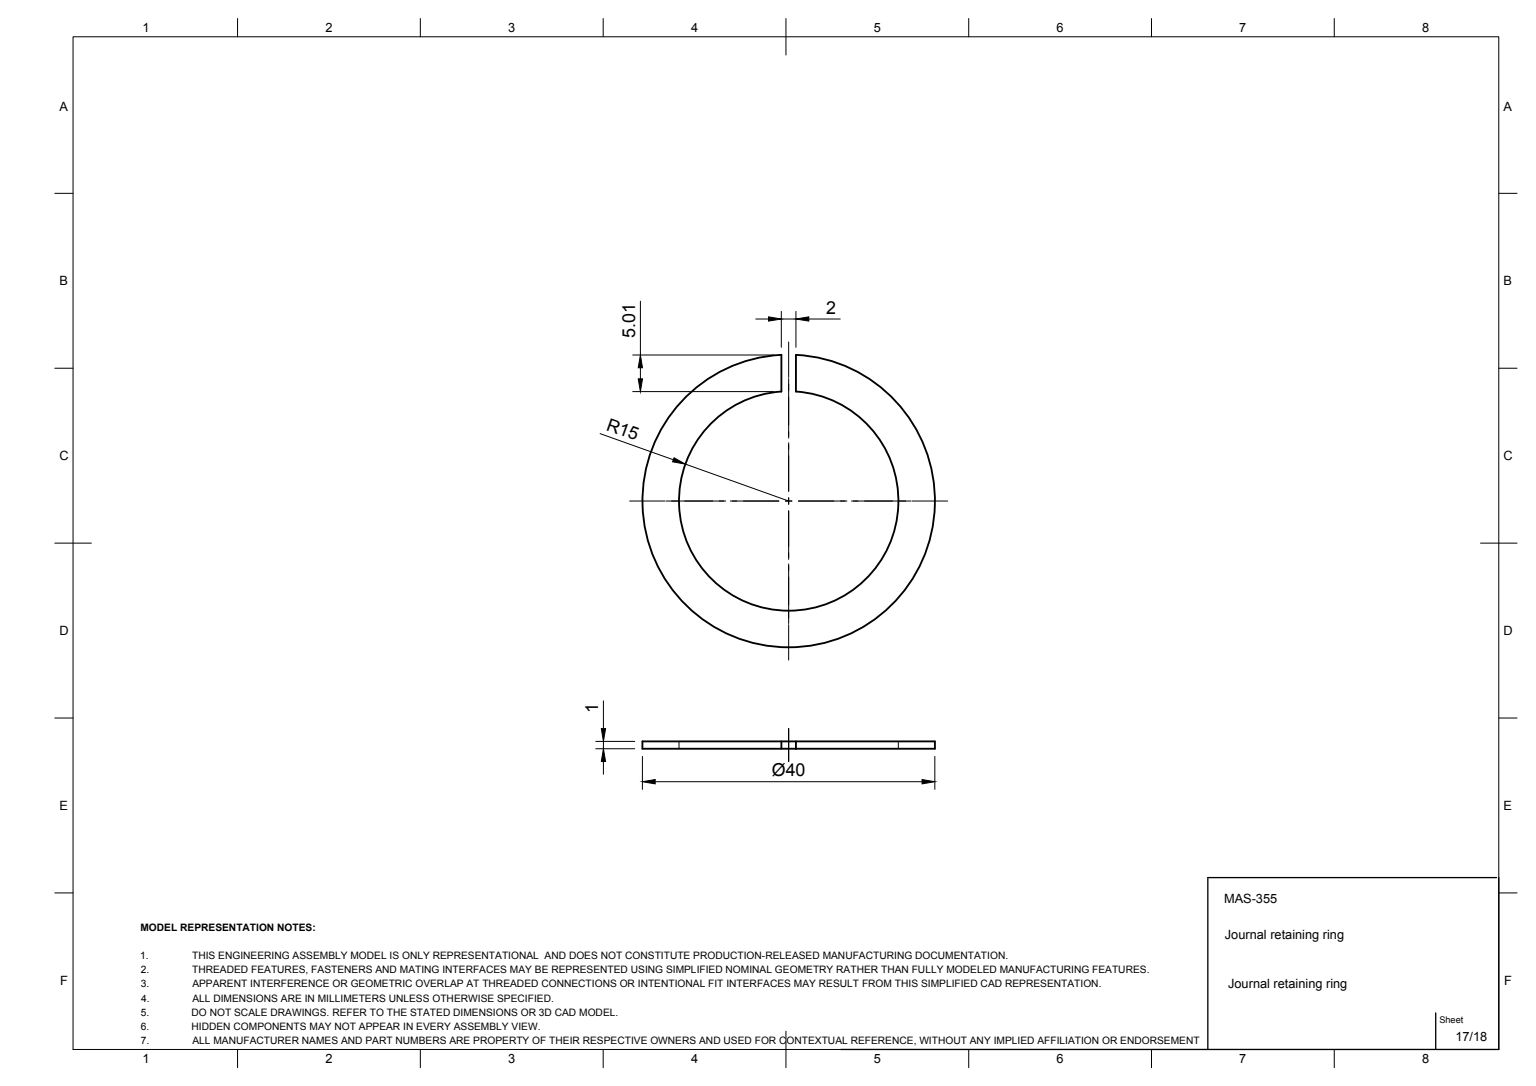
ISO-10303-21;
HEADER;
/* Generated by software containing ST-Developer
 * from STEP Tools, Inc. (www.steptools.com) 
 */

FILE_DESCRIPTION(
/* description */ ('Independent two-stage fixed-ring planetary gearbox,24/24/72 teeth,mod
ule2,20deg involutes,three planets per stage,4:1 x4:1=16:1. Native cut
-space/fillet/pattern tooth profiles derived from reusable gear blanks
; shared sun/planet/ring/carrier parts across both stages. Captured br
onze-journal input/carriers, headed retained planet pins, keyed inters
tage drive and modular keyed output interface. Native ideal gear links
; no torque, precision grade, production backlash/fits, lubrication, s
peed or life rating.'),
/* implementation_level */ '2;1');

FILE_NAME(
/* name */ 'Journal retaining ring.step',
/* time_stamp */ '2026-11-08T19:10:00-08:00',
/* author */ (''),
/* organization */ (''),
/* preprocessor_version */ 'ST-DEVELOPER v20.2',
/* originating_system */ 'Autodesk Translation Framework v15.17.0.0',
/* authorisation */ '');

FILE_SCHEMA (('AUTOMOTIVE_DESIGN { 1 0 10303 214 3 1 1 }'));
ENDSEC;

DATA;
#10=MECHANICAL_DESIGN_GEOMETRIC_PRESENTATION_REPRESENTATION('',(#1180),#259224);
#1140=SHAPE_REPRESENTATION_RELATIONSHIP('SRR','None',#259387,#1160);
#1160=ADVANCED_BREP_SHAPE_REPRESENTATION('',(#1200),#259221);
#1180=STYLED_ITEM('',(#259489),#1200);
#1200=MANIFOLD_SOLID_BREP('Body1',#25167);
#1682=PLANE('',#27160);
#1683=PLANE('',#27161);
#1684=PLANE('',#27162);
#1685=PLANE('',#27169);
#2980=FACE_OUTER_BOUND('',#4439,.T.);
#2981=FACE_OUTER_BOUND('',#4440,.T.);
#2982=FACE_OUTER_BOUND('',#4441,.T.);
#2983=FACE_OUTER_BOUND('',#4442,.T.);
#2984=FACE_OUTER_BOUND('',#4443,.T.);
#2985=FACE_OUTER_BOUND('',#4444,.T.);
#4439=EDGE_LOOP('',(#22742,#22743,#22744,#22745));
#4440=EDGE_LOOP('',(#22746,#22747,#22748,#22749));
#4441=EDGE_LOOP('',(#22750,#22751,#22752,#22753));
#4442=EDGE_LOOP('',(#22754,#22755,#22756,#22757));
#4443=EDGE_LOOP('',(#22758,#22759,#22760,#22761));
#4444=EDGE_LOOP('',(#22762,#22763,#22764,#22765));
#5373=CIRCLE('',#27163,20.);
#5374=CIRCLE('',#27164,15.);
#5375=CIRCLE('',#27166,15.);
#5376=CIRCLE('',#27168,20.);
#7784=LINE('',#256076,#8969);
#7785=LINE('',#256078,#8970);
#7786=LINE('',#256080,#8971);
#7787=LINE('',#256081,#8972);
#7788=LINE('',#256085,#8973);
#7789=LINE('',#256087,#8974);
#7790=LINE('',#256089,#8975);
#7791=LINE('',#256090,#8976);
#8969=VECTOR('',#31991,10.);
#8970=VECTOR('',#31992,10.);
#8971=VECTOR('',#31993,10.);
#8972=VECTOR('',#31994,10.);
#8973=VECTOR('',#31997,10.);
#8974=VECTOR('',#31998,10.);
#8975=VECTOR('',#31999,10.);
#8976=VECTOR('',#32000,10.);
#11485=VERTEX_POINT('',#256074);
#11486=VERTEX_POINT('',#256075);
#11487=VERTEX_POINT('',#256077);
#11488=VERTEX_POINT('',#256079);
#11489=VERTEX_POINT('',#256083);
#11490=VERTEX_POINT('',#256084);
#11491=VERTEX_POINT('',#256086);
#11492=VERTEX_POINT('',#256088);
#15256=EDGE_CURVE('',#11485,#11486,#7784,.T.);
#15257=EDGE_CURVE('',#11487,#11485,#7785,.T.);
#15258=EDGE_CURVE('',#11488,#11487,#7786,.T.);
#15259=EDGE_CURVE('',#11486,#11488,#7787,.T.);
#15260=EDGE_CURVE('',#11489,#11490,#7788,.T.);
#15261=EDGE_CURVE('',#11491,#11489,#7789,.T.);
#15262=EDGE_CURVE('',#11492,#11491,#7790,.T.);
#15263=EDGE_CURVE('',#11490,#11492,#7791,.T.);
#15264=EDGE_CURVE('',#11487,#11492,#5373,.T.);
#15265=EDGE_CURVE('',#11490,#11485,#5374,.T.);
#15266=EDGE_CURVE('',#11489,#11486,#5375,.T.);
#15267=EDGE_CURVE('',#11488,#11491,#5376,.T.);
#22742=ORIENTED_EDGE('',*,*,#15256,.F.);
#22743=ORIENTED_EDGE('',*,*,#15257,.F.);
#22744=ORIENTED_EDGE('',*,*,#15258,.F.);
#22745=ORIENTED_EDGE('',*,*,#15259,.F.);
#22746=ORIENTED_EDGE('',*,*,#15260,.F.);
#22747=ORIENTED_EDGE('',*,*,#15261,.F.);
#22748=ORIENTED_EDGE('',*,*,#15262,.F.);
#22749=ORIENTED_EDGE('',*,*,#15263,.F.);
#22750=ORIENTED_EDGE('',*,*,#15263,.T.);
#22751=ORIENTED_EDGE('',*,*,#15264,.F.);
#22752=ORIENTED_EDGE('',*,*,#15257,.T.);
#22753=ORIENTED_EDGE('',*,*,#15265,.F.);
#22754=ORIENTED_EDGE('',*,*,#15260,.T.);
#22755=ORIENTED_EDGE('',*,*,#15265,.T.);
#22756=ORIENTED_EDGE('',*,*,#15256,.T.);
#22757=ORIENTED_EDGE('',*,*,#15266,.F.);
#22758=ORIENTED_EDGE('',*,*,#15262,.T.);
#22759=ORIENTED_EDGE('',*,*,#15267,.F.);
#22760=ORIENTED_EDGE('',*,*,#15258,.T.);
#22761=ORIENTED_EDGE('',*,*,#15264,.T.);
#22762=ORIENTED_EDGE('',*,*,#15261,.T.);
#22763=ORIENTED_EDGE('',*,*,#15266,.T.);
#22764=ORIENTED_EDGE('',*,*,#15259,.T.);
#22765=ORIENTED_EDGE('',*,*,#15267,.T.);
#23758=CYLINDRICAL_SURFACE('',#27165,15.);
#23759=CYLINDRICAL_SURFACE('',#27167,20.);
#25086=ADVANCED_FACE('',(#2980),#1682,.F.);
#25087=ADVANCED_FACE('',(#2981),#1683,.F.);
#25088=ADVANCED_FACE('',(#2982),#1684,.F.);
#25089=ADVANCED_FACE('',(#2983),#23758,.F.);
#25090=ADVANCED_FACE('',(#2984),#23759,.T.);
#25091=ADVANCED_FACE('',(#2985),#1685,.T.);
#25167=CLOSED_SHELL('',(#25086,#25087,#25088,#25089,#25090,#25091));
#27159=AXIS2_PLACEMENT_3D('',#256072,#31987,#31988);
#27160=AXIS2_PLACEMENT_3D('',#256073,#31989,#31990);
#27161=AXIS2_PLACEMENT_3D('',#256082,#31995,#31996);
#27162=AXIS2_PLACEMENT_3D('',#256091,#32001,#32002);
#27163=AXIS2_PLACEMENT_3D('',#256092,#32003,#32004);
#27164=AXIS2_PLACEMENT_3D('',#256093,#32005,#32006);
#27165=AXIS2_PLACEMENT_3D('',#256094,#32007,#32008);
#27166=AXIS2_PLACEMENT_3D('',#256095,#32009,#32010);
#27167=AXIS2_PLACEMENT_3D('',#256096,#32011,#32012);
#27168=AXIS2_PLACEMENT_3D('',#256097,#32013,#32014);
#27169=AXIS2_PLACEMENT_3D('',#256098,#32015,#32016);
#31987=DIRECTION('axis',(0.,0.,1.));
#31988=DIRECTION('refdir',(1.,0.,0.));
#31989=DIRECTION('center_axis',(-1.,0.,0.));
#31990=DIRECTION('ref_axis',(0.,1.,0.));
#31991=DIRECTION('',(0.,0.,1.));
#31992=DIRECTION('',(0.,-1.,0.));
#31993=DIRECTION('',(0.,0.,-1.));
#31994=DIRECTION('',(0.,1.,0.));
#31995=DIRECTION('center_axis',(1.,0.,0.));
#31996=DIRECTION('ref_axis',(0.,-1.,0.));
#31997=DIRECTION('',(0.,0.,-1.));
#31998=DIRECTION('',(0.,-1.,0.));
#31999=DIRECTION('',(0.,0.,1.));
#32000=DIRECTION('',(0.,1.,0.));
#32001=DIRECTION('center_axis',(0.,0.,1.));
#32002=DIRECTION('ref_axis',(1.,0.,0.));
#32003=DIRECTION('center_axis',(0.,0.,1.));
#32004=DIRECTION('ref_axis',(1.,0.,0.));
#32005=DIRECTION('center_axis',(0.,0.,-1.));
#32006=DIRECTION('ref_axis',(1.,0.,0.));
#32007=DIRECTION('center_axis',(0.,0.,1.));
#32008=DIRECTION('ref_axis',(6.12323399573676E-17,-1.,0.));
#32009=DIRECTION('center_axis',(0.,0.,-1.));
#32010=DIRECTION('ref_axis',(1.,0.,0.));
#32011=DIRECTION('center_axis',(0.,0.,1.));
#32012=DIRECTION('ref_axis',(6.12323399573677E-17,-1.,0.));
#32013=DIRECTION('center_axis',(0.,0.,1.));
#32014=DIRECTION('ref_axis',(1.,0.,0.));
#32015=DIRECTION('center_axis',(0.,0.,1.));
#32016=DIRECTION('ref_axis',(1.,0.,0.));
#256072=CARTESIAN_POINT('',(0.,0.,0.));
#256073=CARTESIAN_POINT('Origin',(-1.,0.,1.));
#256074=CARTESIAN_POINT('',(-1.,14.9666295470958,0.));
#256075=CARTESIAN_POINT('',(-1.,14.9666295470958,1.));
#256076=CARTESIAN_POINT('',(-1.,14.9666295470958,0.));
#256077=CARTESIAN_POINT('',(-1.,19.9749843554382,0.));
#256078=CARTESIAN_POINT('',(-1.,0.,0.));
#256079=CARTESIAN_POINT('',(-1.,19.9749843554382,1.));
#256080=CARTESIAN_POINT('',(-1.,19.9749843554382,0.));
#256081=CARTESIAN_POINT('',(-1.,0.,1.));
#256082=CARTESIAN_POINT('Origin',(1.,40.,1.));
#256083=CARTESIAN_POINT('',(1.,14.9666295470958,1.));
#256084=CARTESIAN_POINT('',(1.,14.9666295470958,0.));
#256085=CARTESIAN_POINT('',(1.,14.9666295470958,0.));
#256086=CARTESIAN_POINT('',(1.,19.9749843554382,1.));
#256087=CARTESIAN_POINT('',(1.,20.,1.));
#256088=CARTESIAN_POINT('',(1.,19.9749843554382,0.));
#256089=CARTESIAN_POINT('',(1.,19.9749843554382,0.));
#256090=CARTESIAN_POINT('',(1.,20.,0.));
#256091=CARTESIAN_POINT('Origin',(0.,0.,0.));
#256092=CARTESIAN_POINT('Origin',(0.,0.,0.));
#256093=CARTESIAN_POINT('Origin',(0.,0.,0.));
#256094=CARTESIAN_POINT('Origin',(0.,0.,0.));
#256095=CARTESIAN_POINT('Origin',(0.,0.,1.));
#256096=CARTESIAN_POINT('Origin',(0.,0.,0.));
#256097=CARTESIAN_POINT('Origin',(0.,0.,1.));
#256098=CARTESIAN_POINT('Origin',(0.,0.,1.));
#259199=UNCERTAINTY_MEASURE_WITH_UNIT(LENGTH_MEASURE(0.01),#259225,
'DISTANCE_ACCURACY_VALUE',
'Maximum model space distance between geometric entities at asserted c
onnectivities');
#259202=UNCERTAINTY_MEASURE_WITH_UNIT(LENGTH_MEASURE(0.01),#259225,
'DISTANCE_ACCURACY_VALUE',
'Maximum model space distance between geometric entities at asserted c
onnectivities');
#259221=(
GEOMETRIC_REPRESENTATION_CONTEXT(3)
GLOBAL_UNCERTAINTY_ASSIGNED_CONTEXT((#259199))
GLOBAL_UNIT_ASSIGNED_CONTEXT((#259225,#259227,#259228))
REPRESENTATION_CONTEXT('','3D')
);
#259224=(
GEOMETRIC_REPRESENTATION_CONTEXT(3)
GLOBAL_UNCERTAINTY_ASSIGNED_CONTEXT((#259202))
GLOBAL_UNIT_ASSIGNED_CONTEXT((#259225,#259227,#259228))
REPRESENTATION_CONTEXT('','3D')
);
#259225=(
LENGTH_UNIT()
NAMED_UNIT(*)
SI_UNIT(.MILLI.,.METRE.)
);
#259227=(
NAMED_UNIT(*)
PLANE_ANGLE_UNIT()
SI_UNIT($,.RADIAN.)
);
#259228=(
NAMED_UNIT(*)
SI_UNIT($,.STERADIAN.)
SOLID_ANGLE_UNIT()
);
#259247=SHAPE_DEFINITION_REPRESENTATION(#259268,#259387);
#259268=PRODUCT_DEFINITION_SHAPE('',$,#259409);
#259387=SHAPE_REPRESENTATION('',(#27159),#259221);
#259390=PRODUCT_DEFINITION_CONTEXT('part definition',#259455,'design');
#259409=PRODUCT_DEFINITION('Journal retaining ring',
'Journal retaining ring',#259430,#259390);
#259430=PRODUCT_DEFINITION_FORMATION('',$,#259475);
#259455=APPLICATION_CONTEXT(
'Core Data for Automotive Mechanical Design Process');
#259456=PRODUCT_CONTEXT('part definition',#259455,'mechanical');
#259475=PRODUCT('Journal retaining ring','Journal retaining ring',$,(#259456));
#259489=PRESENTATION_STYLE_ASSIGNMENT((#259504));
#259504=SURFACE_STYLE_USAGE(.BOTH.,#259519);
#259519=SURFACE_SIDE_STYLE('',(#259534));
#259534=SURFACE_STYLE_FILL_AREA(#259549);
#259549=FILL_AREA_STYLE('Dark gray',(#259564));
#259564=FILL_AREA_STYLE_COLOUR('Dark gray',#259579);
#259579=COLOUR_RGB('Dark gray',0.250980392156863,0.282352941176471,0.32156862745098);
ENDSEC;
END-ISO-10303-21;
